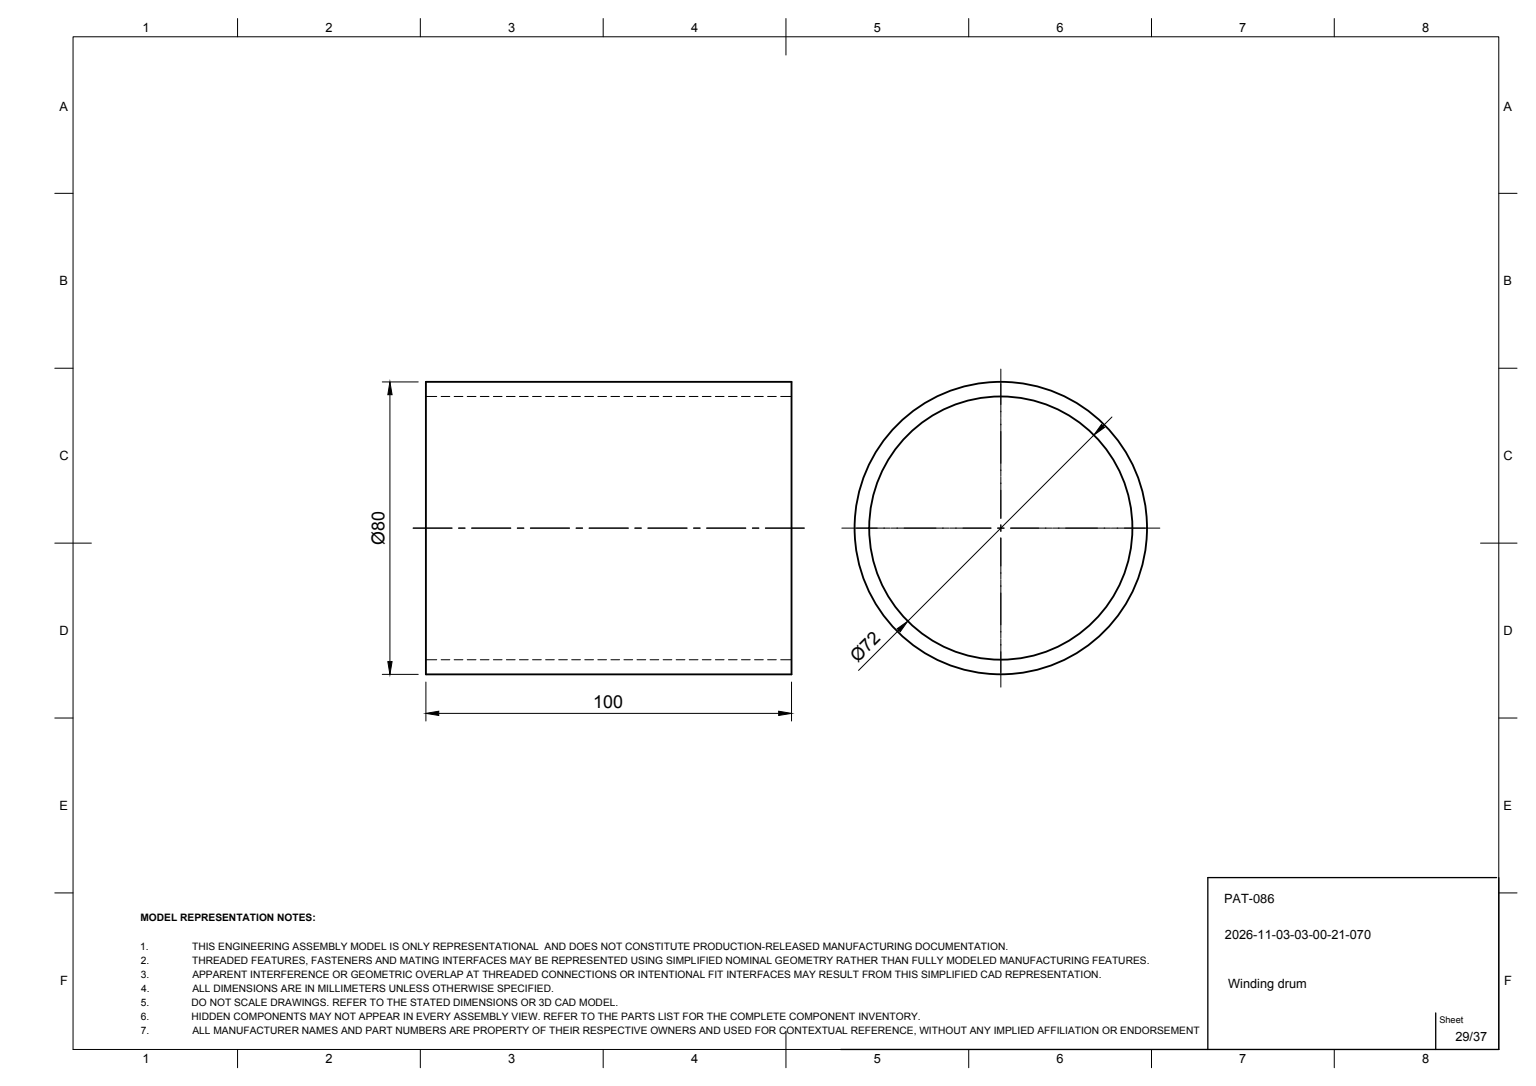
ISO-10303-21;
HEADER;
/* Generated by software containing ST-Developer
 * from STEP Tools, Inc. (www.steptools.com) 
 */

FILE_DESCRIPTION(
/* description */ ('Ratchet and pawl hand winch drum'),
/* implementation_level */ '2;1');

FILE_NAME(
/* name */ 'Winding drum.step',
/* time_stamp */ '2026-10-27T12:42:58-07:00',
/* author */ (''),
/* organization */ (''),
/* preprocessor_version */ 'ST-DEVELOPER v20.2',
/* originating_system */ 'Autodesk Translation Framework v15.17.0.0',
/* authorisation */ '');

FILE_SCHEMA (('AUTOMOTIVE_DESIGN { 1 0 10303 214 3 1 1 }'));
ENDSEC;

DATA;
#10=MECHANICAL_DESIGN_GEOMETRIC_PRESENTATION_REPRESENTATION('',(#413),#11801);
#344=SHAPE_REPRESENTATION_RELATIONSHIP('SRR','None',#11972,#378);
#378=ADVANCED_BREP_SHAPE_REPRESENTATION('',(#446),#11789);
#413=STYLED_ITEM('',(#12227),#446);
#446=MANIFOLD_SOLID_BREP('Body1',#6292);
#572=FACE_BOUND('',#1535,.T.);
#573=FACE_BOUND('',#1537,.T.);
#736=PLANE('',#7093);
#737=PLANE('',#7094);
#1060=FACE_OUTER_BOUND('',#1532,.T.);
#1061=FACE_OUTER_BOUND('',#1533,.T.);
#1062=FACE_OUTER_BOUND('',#1534,.T.);
#1063=FACE_OUTER_BOUND('',#1536,.T.);
#1532=EDGE_LOOP('',(#5171,#5172,#5173,#5174));
#1533=EDGE_LOOP('',(#5175,#5176,#5177,#5178));
#1534=EDGE_LOOP('',(#5179));
#1535=EDGE_LOOP('',(#5180));
#1536=EDGE_LOOP('',(#5181));
#1537=EDGE_LOOP('',(#5182));
#1969=LINE('',#10785,#2480);
#1970=LINE('',#10791,#2481);
#2480=VECTOR('',#8450,3.6);
#2481=VECTOR('',#8457,4.);
#2877=CIRCLE('',#7088,3.6);
#2878=CIRCLE('',#7089,3.6);
#2879=CIRCLE('',#7091,4.);
#2880=CIRCLE('',#7092,4.);
#3256=VERTEX_POINT('',#10782);
#3257=VERTEX_POINT('',#10784);
#3258=VERTEX_POINT('',#10788);
#3259=VERTEX_POINT('',#10790);
#3929=EDGE_CURVE('',#3256,#3256,#2877,.T.);
#3930=EDGE_CURVE('',#3256,#3257,#1969,.T.);
#3931=EDGE_CURVE('',#3257,#3257,#2878,.T.);
#3932=EDGE_CURVE('',#3258,#3258,#2879,.T.);
#3933=EDGE_CURVE('',#3258,#3259,#1970,.T.);
#3934=EDGE_CURVE('',#3259,#3259,#2880,.T.);
#5171=ORIENTED_EDGE('',*,*,#3929,.F.);
#5172=ORIENTED_EDGE('',*,*,#3930,.T.);
#5173=ORIENTED_EDGE('',*,*,#3931,.T.);
#5174=ORIENTED_EDGE('',*,*,#3930,.F.);
#5175=ORIENTED_EDGE('',*,*,#3932,.F.);
#5176=ORIENTED_EDGE('',*,*,#3933,.T.);
#5177=ORIENTED_EDGE('',*,*,#3934,.T.);
#5178=ORIENTED_EDGE('',*,*,#3933,.F.);
#5179=ORIENTED_EDGE('',*,*,#3932,.T.);
#5180=ORIENTED_EDGE('',*,*,#3929,.T.);
#5181=ORIENTED_EDGE('',*,*,#3934,.F.);
#5182=ORIENTED_EDGE('',*,*,#3931,.F.);
#5884=CYLINDRICAL_SURFACE('',#7087,3.6);
#5885=CYLINDRICAL_SURFACE('',#7090,4.);
#6130=ADVANCED_FACE('',(#1060),#5884,.F.);
#6131=ADVANCED_FACE('',(#1061),#5885,.T.);
#6132=ADVANCED_FACE('',(#1062,#572),#736,.T.);
#6133=ADVANCED_FACE('',(#1063,#573),#737,.F.);
#6292=CLOSED_SHELL('',(#6130,#6131,#6132,#6133));
#7086=AXIS2_PLACEMENT_3D('',#10780,#8444,#8445);
#7087=AXIS2_PLACEMENT_3D('',#10781,#8446,#8447);
#7088=AXIS2_PLACEMENT_3D('',#10783,#8448,#8449);
#7089=AXIS2_PLACEMENT_3D('',#10786,#8451,#8452);
#7090=AXIS2_PLACEMENT_3D('',#10787,#8453,#8454);
#7091=AXIS2_PLACEMENT_3D('',#10789,#8455,#8456);
#7092=AXIS2_PLACEMENT_3D('',#10792,#8458,#8459);
#7093=AXIS2_PLACEMENT_3D('',#10793,#8460,#8461);
#7094=AXIS2_PLACEMENT_3D('',#10794,#8462,#8463);
#8444=DIRECTION('axis',(0.,0.,1.));
#8445=DIRECTION('refdir',(1.,0.,0.));
#8446=DIRECTION('center_axis',(0.,1.,0.));
#8447=DIRECTION('ref_axis',(1.,0.,0.));
#8448=DIRECTION('center_axis',(0.,-1.,0.));
#8449=DIRECTION('ref_axis',(1.,0.,0.));
#8450=DIRECTION('',(0.,-1.,0.));
#8451=DIRECTION('center_axis',(0.,-1.,0.));
#8452=DIRECTION('ref_axis',(1.,0.,0.));
#8453=DIRECTION('center_axis',(0.,1.,0.));
#8454=DIRECTION('ref_axis',(1.,0.,0.));
#8455=DIRECTION('center_axis',(0.,1.,0.));
#8456=DIRECTION('ref_axis',(1.,0.,0.));
#8457=DIRECTION('',(0.,-1.,0.));
#8458=DIRECTION('center_axis',(0.,1.,0.));
#8459=DIRECTION('ref_axis',(1.,0.,0.));
#8460=DIRECTION('center_axis',(0.,1.,0.));
#8461=DIRECTION('ref_axis',(1.,0.,0.));
#8462=DIRECTION('center_axis',(0.,1.,0.));
#8463=DIRECTION('ref_axis',(1.,0.,0.));
#10780=CARTESIAN_POINT('',(0.,0.,0.));
#10781=CARTESIAN_POINT('Origin',(0.,3.,6.53));
#10782=CARTESIAN_POINT('',(-3.6,13.,6.53));
#10783=CARTESIAN_POINT('Origin',(0.,13.,6.53));
#10784=CARTESIAN_POINT('',(-3.6,3.,6.53));
#10785=CARTESIAN_POINT('',(-3.6,3.,6.53));
#10786=CARTESIAN_POINT('Origin',(0.,3.,6.53));
#10787=CARTESIAN_POINT('Origin',(0.,3.,6.53));
#10788=CARTESIAN_POINT('',(-4.,13.,6.53));
#10789=CARTESIAN_POINT('Origin',(0.,13.,6.53));
#10790=CARTESIAN_POINT('',(-4.,3.,6.53));
#10791=CARTESIAN_POINT('',(-4.,3.,6.53));
#10792=CARTESIAN_POINT('Origin',(0.,3.,6.53));
#10793=CARTESIAN_POINT('Origin',(0.,13.,6.53));
#10794=CARTESIAN_POINT('Origin',(0.,3.,6.53));
#11749=UNCERTAINTY_MEASURE_WITH_UNIT(LENGTH_MEASURE(0.001),#11802,
'DISTANCE_ACCURACY_VALUE',
'Maximum model space distance between geometric entities at asserted c
onnectivities');
#11761=UNCERTAINTY_MEASURE_WITH_UNIT(LENGTH_MEASURE(0.001),#11802,
'DISTANCE_ACCURACY_VALUE',
'Maximum model space distance between geometric entities at asserted c
onnectivities');
#11789=(
GEOMETRIC_REPRESENTATION_CONTEXT(3)
GLOBAL_UNCERTAINTY_ASSIGNED_CONTEXT((#11749))
GLOBAL_UNIT_ASSIGNED_CONTEXT((#11802,#11804,#11805))
REPRESENTATION_CONTEXT('','3D')
);
#11801=(
GEOMETRIC_REPRESENTATION_CONTEXT(3)
GLOBAL_UNCERTAINTY_ASSIGNED_CONTEXT((#11761))
GLOBAL_UNIT_ASSIGNED_CONTEXT((#11802,#11804,#11805))
REPRESENTATION_CONTEXT('','3D')
);
#11802=(
LENGTH_UNIT()
NAMED_UNIT(*)
SI_UNIT(.CENTI.,.METRE.)
);
#11804=(
NAMED_UNIT(*)
PLANE_ANGLE_UNIT()
SI_UNIT($,.RADIAN.)
);
#11805=(
NAMED_UNIT(*)
SI_UNIT($,.STERADIAN.)
SOLID_ANGLE_UNIT()
);
#11833=SHAPE_DEFINITION_REPRESENTATION(#11874,#11972);
#11874=PRODUCT_DEFINITION_SHAPE('',$,#12012);
#11972=SHAPE_REPRESENTATION('',(#7086),#11789);
#11984=PRODUCT_DEFINITION_CONTEXT('part definition',#12103,'design');
#12012=PRODUCT_DEFINITION('Winding drum','Winding drum',#12051,#11984);
#12051=PRODUCT_DEFINITION_FORMATION('',$,#12132);
#12103=APPLICATION_CONTEXT(
'Core Data for Automotive Mechanical Design Process');
#12104=PRODUCT_CONTEXT('part definition',#12103,'mechanical');
#12132=PRODUCT('Winding drum','Winding drum','Winding drum',(#12104));
#12221=COLOUR_RGB('Off White',0.89,0.88,0.83);
#12222=FILL_AREA_STYLE_COLOUR('',#12221);
#12223=FILL_AREA_STYLE('',(#12222));
#12224=SURFACE_STYLE_FILL_AREA(#12223);
#12225=SURFACE_SIDE_STYLE('',(#12224));
#12226=SURFACE_STYLE_USAGE(.BOTH.,#12225);
#12227=PRESENTATION_STYLE_ASSIGNMENT((#12226));
ENDSEC;
END-ISO-10303-21;
